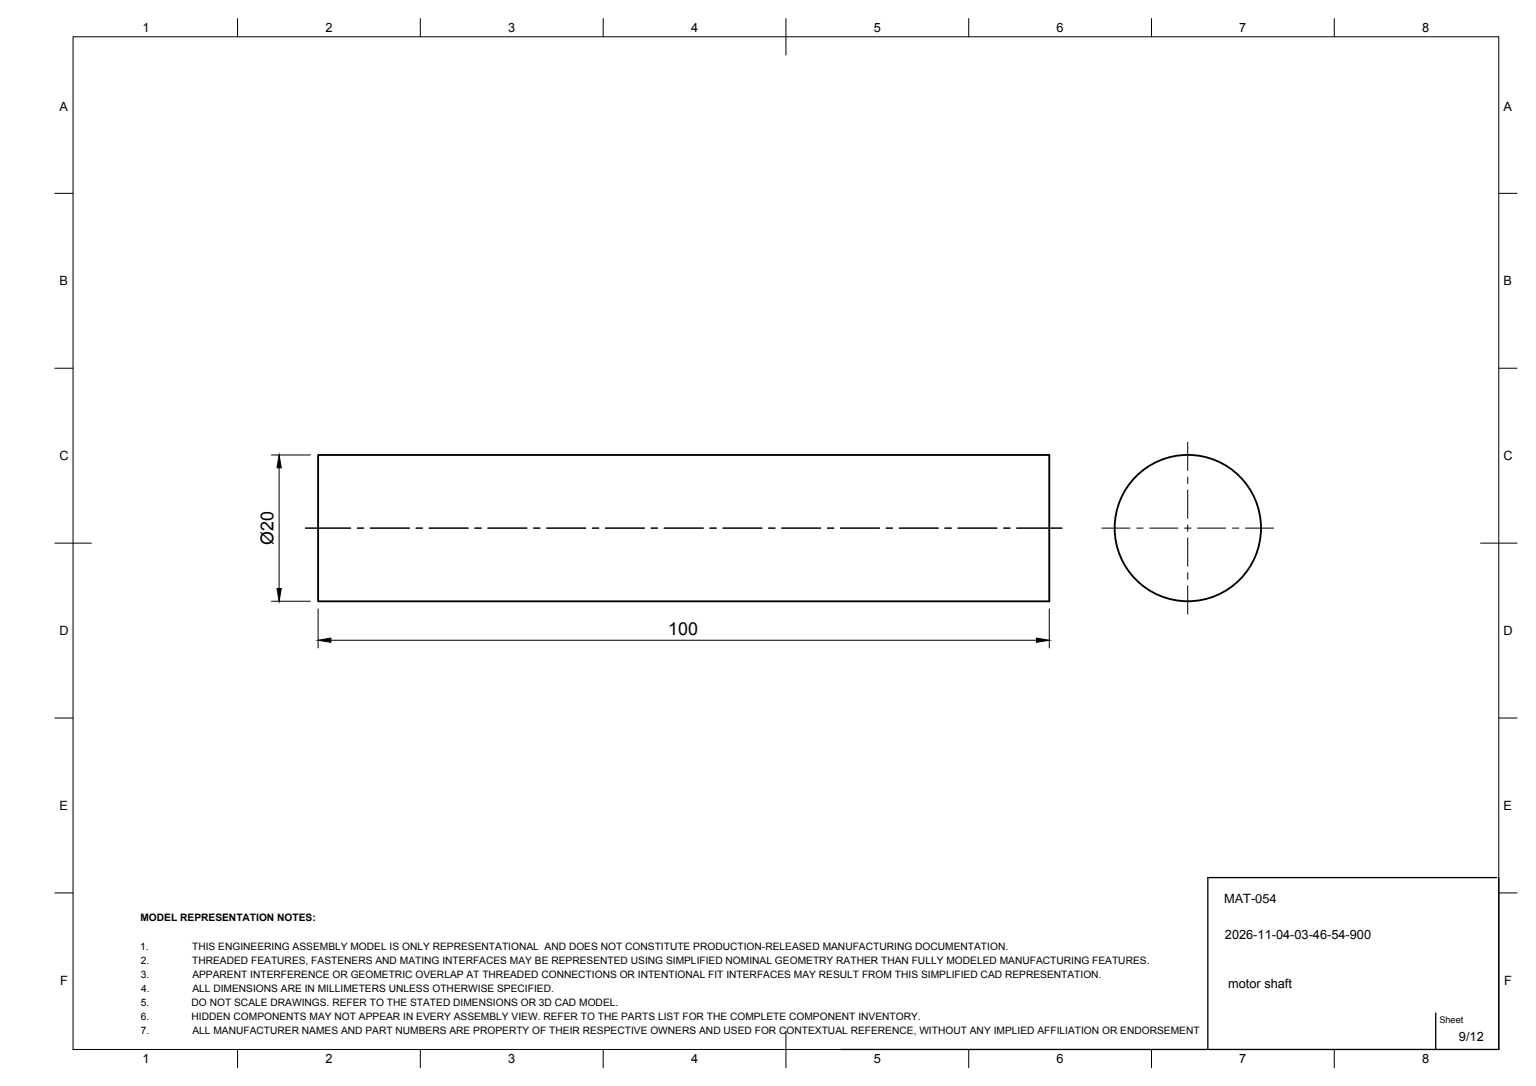
ISO-10303-21;
HEADER;
FILE_DESCRIPTION (('STEP AP214'),
    '1' );
FILE_NAME ('motor shaft.step',
    '2026-10-21T17:50:41',
    ( '' ),
    ( '' ),
    'SwSTEP 2.0',
    'SolidWorks 2026',
    '' );
FILE_SCHEMA (( 'AUTOMOTIVE_DESIGN' ));
ENDSEC;

DATA;
#3=DIRECTION ( 'NONE',  ( 0.000000000000000000, 1.000000000000000000, 0.000000000000000000 ) ) ;
#225=DIRECTION ( 'NONE',  ( 0.000000000000000000, 0.000000000000000000, 1.000000000000000000 ) ) ;
#325=EDGE_CURVE ( 'NONE', #23614, #34805, #30448, .T. ) ;
#547=APPLICATION_CONTEXT ( 'automotive_design' ) ;
#600=AXIS2_PLACEMENT_3D ( 'NONE', #10978, #16688, #29670 ) ;
#1566=ORIENTED_EDGE ( 'NONE', *, *, #325, .T. ) ;
#2200=DIRECTION ( 'NONE',  ( 0.000000000000000000, 0.000000000000000000, 1.000000000000000000 ) ) ;
#2586=ORIENTED_EDGE ( 'NONE', *, *, #23860, .T. ) ;
#2881=DIRECTION ( 'NONE',  ( 0.000000000000000000, 1.000000000000000000, 0.000000000000000000 ) ) ;
#2917=AXIS2_PLACEMENT_3D ( 'NONE', #19073, #32391, #13546 ) ;
#4429=ADVANCED_FACE ( 'NONE', ( #23028 ), #33880, .T. ) ;
#4458=( NAMED_UNIT ( * ) PLANE_ANGLE_UNIT ( ) SI_UNIT ( $, .RADIAN. ) );
#5868=PRODUCT_CONTEXT ( 'NONE', #547, 'mechanical' ) ;
#6007=EDGE_LOOP ( 'NONE', ( #2586, #1566 ) ) ;
#6174=FACE_OUTER_BOUND ( 'NONE', #12972, .T. ) ;
#6802=DIRECTION ( 'NONE',  ( 0.000000000000000000, 0.000000000000000000, 1.000000000000000000 ) ) ;
#6830=ORIENTED_EDGE ( 'NONE', *, *, #9360, .T. ) ;
#7370=UNCERTAINTY_MEASURE_WITH_UNIT (LENGTH_MEASURE( 1.000000000000000082E-05 ), #24179, 'distance_accuracy_value', 'NONE');
#7616=CARTESIAN_POINT ( 'NONE',  ( 0.000000000000000000, 49.99999999999999289, -9.999999999999998224 ) ) ;
#7626=VECTOR ( 'NONE', #29268, 1000.000000000000000 ) ;
#7803=( NAMED_UNIT ( * ) SI_UNIT ( $, .STERADIAN. ) SOLID_ANGLE_UNIT ( ) );
#8023=CIRCLE ( 'NONE', #2917, 9.999999999999998224 ) ;
#8681=DIRECTION ( 'NONE',  ( 0.000000000000000000, 1.000000000000000000, 0.000000000000000000 ) ) ;
#9360=EDGE_CURVE ( 'NONE', #29353, #16028, #26584, .T. ) ;
#9405=EDGE_CURVE ( 'NONE', #23614, #29353, #21713, .T. ) ;
#9663=DIRECTION ( 'NONE',  ( 0.000000000000000000, 1.000000000000000000, 0.000000000000000000 ) ) ;
#9735=AXIS2_PLACEMENT_3D ( 'NONE', #34546, #29388, #15343 ) ;
#10049=CARTESIAN_POINT ( 'NONE',  ( 0.000000000000000000, 49.99999999999999289, -9.999999999999998224 ) ) ;
#10060=MANIFOLD_SOLID_BREP ( 'Boss-Extrude1', #33097 ) ;
#10978=CARTESIAN_POINT ( 'NONE',  ( 0.000000000000000000, 49.99999999999999289, 0.000000000000000000 ) ) ;
#11651=CARTESIAN_POINT ( 'NONE',  ( 0.000000000000000000, 49.99999999999999289, 0.000000000000000000 ) ) ;
#11880=CARTESIAN_POINT ( 'NONE',  ( 0.000000000000000000, -49.99999999999999289, -9.999999999999998224 ) ) ;
#11977=CARTESIAN_POINT ( 'NONE',  ( 1.224646799147352862E-15, 49.99999999999999289, 9.999999999999998224 ) ) ;
#12177=DIRECTION ( 'NONE',  ( 0.000000000000000000, 1.000000000000000000, 0.000000000000000000 ) ) ;
#12676=FACE_OUTER_BOUND ( 'NONE', #15104, .T. ) ;
#12835=ORIENTED_EDGE ( 'NONE', *, *, #17849, .F. ) ;
#12972=EDGE_LOOP ( 'NONE', ( #31313, #14636 ) ) ;
#13073=DIRECTION ( 'NONE',  ( 1.000000000000000000, 0.000000000000000000, 0.000000000000000000 ) ) ;
#13488=ADVANCED_FACE ( 'NONE', ( #6174 ), #28435, .F. ) ;
#13546=DIRECTION ( 'NONE',  ( 0.000000000000000000, 0.000000000000000000, 1.000000000000000000 ) ) ;
#13758=CARTESIAN_POINT ( 'NONE',  ( 0.000000000000000000, 49.99999999999999289, 0.000000000000000000 ) ) ;
#14046=PRODUCT ( 'motor shaft', 'motor shaft', '', ( #5868 ) ) ;
#14245=ORIENTED_EDGE ( 'NONE', *, *, #17849, .T. ) ;
#14307=ORIENTED_EDGE ( 'NONE', *, *, #9405, .F. ) ;
#14636=ORIENTED_EDGE ( 'NONE', *, *, #9360, .F. ) ;
#15104=EDGE_LOOP ( 'NONE', ( #14307, #23131, #14245, #27576 ) ) ;
#15295=EDGE_CURVE ( 'NONE', #16028, #29353, #31888, .T. ) ;
#15303=( GEOMETRIC_REPRESENTATION_CONTEXT ( 3 ) GLOBAL_UNCERTAINTY_ASSIGNED_CONTEXT ( ( #7370 ) ) GLOBAL_UNIT_ASSIGNED_CONTEXT ( ( #24179, #32011, #7803 ) ) REPRESENTATION_CONTEXT ( 'NONE', 'WORKASPACE' ) );
#15343=DIRECTION ( 'NONE',  ( 0.000000000000000000, 0.000000000000000000, -1.000000000000000000 ) ) ;
#15348=( NAMED_UNIT ( * ) SI_UNIT ( $, .STERADIAN. ) SOLID_ANGLE_UNIT ( ) );
#15819=AXIS2_PLACEMENT_3D ( 'NONE', #30082, #3, #24726 ) ;
#15847=ADVANCED_FACE ( 'NONE', ( #30192 ), #32857, .T. ) ;
#16028=VERTEX_POINT ( 'NONE', #11880 ) ;
#16688=DIRECTION ( 'NONE',  ( -0.000000000000000000, -1.000000000000000000, -0.000000000000000000 ) ) ;
#16831=AXIS2_PLACEMENT_3D ( 'NONE', #13758, #2881, #225 ) ;
#17780=PRODUCT_DEFINITION_SHAPE ( 'NONE', 'NONE',  #18183 ) ;
#17849=EDGE_CURVE ( 'NONE', #34805, #16028, #32278, .T. ) ;
#18183=PRODUCT_DEFINITION ( 'UNKNOWN', '', #30925, #18560 ) ;
#18221=CARTESIAN_POINT ( 'NONE',  ( 1.224646799147352862E-15, -49.99999999999999289, 9.999999999999998224 ) ) ;
#18560=PRODUCT_DEFINITION_CONTEXT ( 'detailed design', #29647, 'design' ) ;
#18659=VECTOR ( 'NONE', #33091, 1000.000000000000000 ) ;
#19073=CARTESIAN_POINT ( 'NONE',  ( 0.000000000000000000, 49.99999999999999289, 0.000000000000000000 ) ) ;
#19498=ADVANCED_BREP_SHAPE_REPRESENTATION ( '', ( #10060, #28566 ), #30284 ) ;
#19557=DIRECTION ( 'NONE',  ( 0.000000000000000000, -0.000000000000000000, 1.000000000000000000 ) ) ;
#19954=ORIENTED_EDGE ( 'NONE', *, *, #325, .F. ) ;
#20360=DIRECTION ( 'NONE',  ( 0.000000000000000000, -0.000000000000000000, 1.000000000000000000 ) ) ;
#21713=LINE ( 'NONE', #24901, #18659 ) ;
#22158=AXIS2_PLACEMENT_3D ( 'NONE', #22215, #8681, #19557 ) ;
#22215=CARTESIAN_POINT ( 'NONE',  ( 0.000000000000000000, -49.99999999999999289, 0.000000000000000000 ) ) ;
#23028=FACE_OUTER_BOUND ( 'NONE', #6007, .T. ) ;
#23131=ORIENTED_EDGE ( 'NONE', *, *, #23860, .F. ) ;
#23139=UNCERTAINTY_MEASURE_WITH_UNIT (LENGTH_MEASURE( 1.000000000000000082E-05 ), #25664, 'distance_accuracy_value', 'NONE');
#23614=VERTEX_POINT ( 'NONE', #11977 ) ;
#23699=ADVANCED_FACE ( 'NONE', ( #12676 ), #26530, .T. ) ;
#23860=EDGE_CURVE ( 'NONE', #34805, #23614, #8023, .T. ) ;
#24179=( LENGTH_UNIT ( ) NAMED_UNIT ( * ) SI_UNIT ( .MILLI., .METRE. ) );
#24562=SHAPE_DEFINITION_REPRESENTATION ( #17780, #29156 ) ;
#24726=DIRECTION ( 'NONE',  ( 0.000000000000000000, 0.000000000000000000, 1.000000000000000000 ) ) ;
#24901=CARTESIAN_POINT ( 'NONE',  ( 1.224646799147352862E-15, 49.99999999999999289, 9.999999999999998224 ) ) ;
#25664=( LENGTH_UNIT ( ) NAMED_UNIT ( * ) SI_UNIT ( .MILLI., .METRE. ) );
#26362=SHAPE_REPRESENTATION_RELATIONSHIP ( 'NONE' , 'NONE' ,  #29156, #19498 ) ;
#26530=CYLINDRICAL_SURFACE ( 'NONE', #9735, 9.999999999999998224 ) ;
#26579=CARTESIAN_POINT ( 'NONE',  ( 0.000000000000000000, 0.000000000000000000, 0.000000000000000000 ) ) ;
#26584=CIRCLE ( 'NONE', #15819, 9.999999999999998224 ) ;
#27238=AXIS2_PLACEMENT_3D ( 'NONE', #11651, #9663, #20360 ) ;
#27576=ORIENTED_EDGE ( 'NONE', *, *, #15295, .T. ) ;
#28328=MECHANICAL_DESIGN_GEOMETRIC_PRESENTATION_REPRESENTATION('',(#31172),#15303);
#28435=PLANE ( 'NONE',  #22158 ) ;
#28566=AXIS2_PLACEMENT_3D ( 'NONE', #26579, #2200, #13073 ) ;
#29075=AXIS2_PLACEMENT_3D ( 'NONE', #31712, #12177, #6802 ) ;
#29156=SHAPE_REPRESENTATION ( 'motor shaft', ( #28566 ), #30284 ) ;
#29268=DIRECTION ( 'NONE',  ( -0.000000000000000000, -1.000000000000000000, -0.000000000000000000 ) ) ;
#29353=VERTEX_POINT ( 'NONE', #18221 ) ;
#29388=DIRECTION ( 'NONE',  ( -0.000000000000000000, -1.000000000000000000, -0.000000000000000000 ) ) ;
#29647=APPLICATION_CONTEXT ( 'automotive_design' ) ;
#29670=DIRECTION ( 'NONE',  ( 0.000000000000000000, 0.000000000000000000, -1.000000000000000000 ) ) ;
#30082=CARTESIAN_POINT ( 'NONE',  ( 0.000000000000000000, -49.99999999999999289, 0.000000000000000000 ) ) ;
#30192=FACE_OUTER_BOUND ( 'NONE', #32156, .T. ) ;
#30284=( GEOMETRIC_REPRESENTATION_CONTEXT ( 3 ) GLOBAL_UNCERTAINTY_ASSIGNED_CONTEXT ( ( #23139 ) ) GLOBAL_UNIT_ASSIGNED_CONTEXT ( ( #25664, #4458, #15348 ) ) REPRESENTATION_CONTEXT ( 'NONE', 'WORKASPACE' ) );
#30303=ORIENTED_EDGE ( 'NONE', *, *, #9405, .T. ) ;
#30448=CIRCLE ( 'NONE', #16831, 9.999999999999998224 ) ;
#30925=PRODUCT_DEFINITION_FORMATION_WITH_SPECIFIED_SOURCE ( 'ANY', '', #14046, .NOT_KNOWN. ) ;
#31172=STYLED_ITEM('',(#35275),#10060);
#31313=ORIENTED_EDGE ( 'NONE', *, *, #15295, .F. ) ;
#31712=CARTESIAN_POINT ( 'NONE',  ( 0.000000000000000000, -49.99999999999999289, 0.000000000000000000 ) ) ;
#31888=CIRCLE ( 'NONE', #29075, 9.999999999999998224 ) ;
#32011=( NAMED_UNIT ( * ) PLANE_ANGLE_UNIT ( ) SI_UNIT ( $, .RADIAN. ) );
#32156=EDGE_LOOP ( 'NONE', ( #19954, #30303, #6830, #12835 ) ) ;
#32278=LINE ( 'NONE', #10049, #7626 ) ;
#32391=DIRECTION ( 'NONE',  ( 0.000000000000000000, 1.000000000000000000, 0.000000000000000000 ) ) ;
#32857=CYLINDRICAL_SURFACE ( 'NONE', #600, 9.999999999999998224 ) ;
#33091=DIRECTION ( 'NONE',  ( -0.000000000000000000, -1.000000000000000000, -0.000000000000000000 ) ) ;
#33097=CLOSED_SHELL ( 'NONE', ( #15847, #23699, #4429, #13488 ) ) ;
#33880=PLANE ( 'NONE',  #27238 ) ;
#34546=CARTESIAN_POINT ( 'NONE',  ( 0.000000000000000000, 49.99999999999999289, 0.000000000000000000 ) ) ;
#34805=VERTEX_POINT ( 'NONE', #7616 ) ;
#35269=COLOUR_RGB('Grey',0.48,0.52,0.57);
#35270=FILL_AREA_STYLE_COLOUR('',#35269);
#35271=FILL_AREA_STYLE('',(#35270));
#35272=SURFACE_STYLE_FILL_AREA(#35271);
#35273=SURFACE_SIDE_STYLE('',(#35272));
#35274=SURFACE_STYLE_USAGE(.BOTH.,#35273);
#35275=PRESENTATION_STYLE_ASSIGNMENT((#35274));
ENDSEC;
END-ISO-10303-21;
